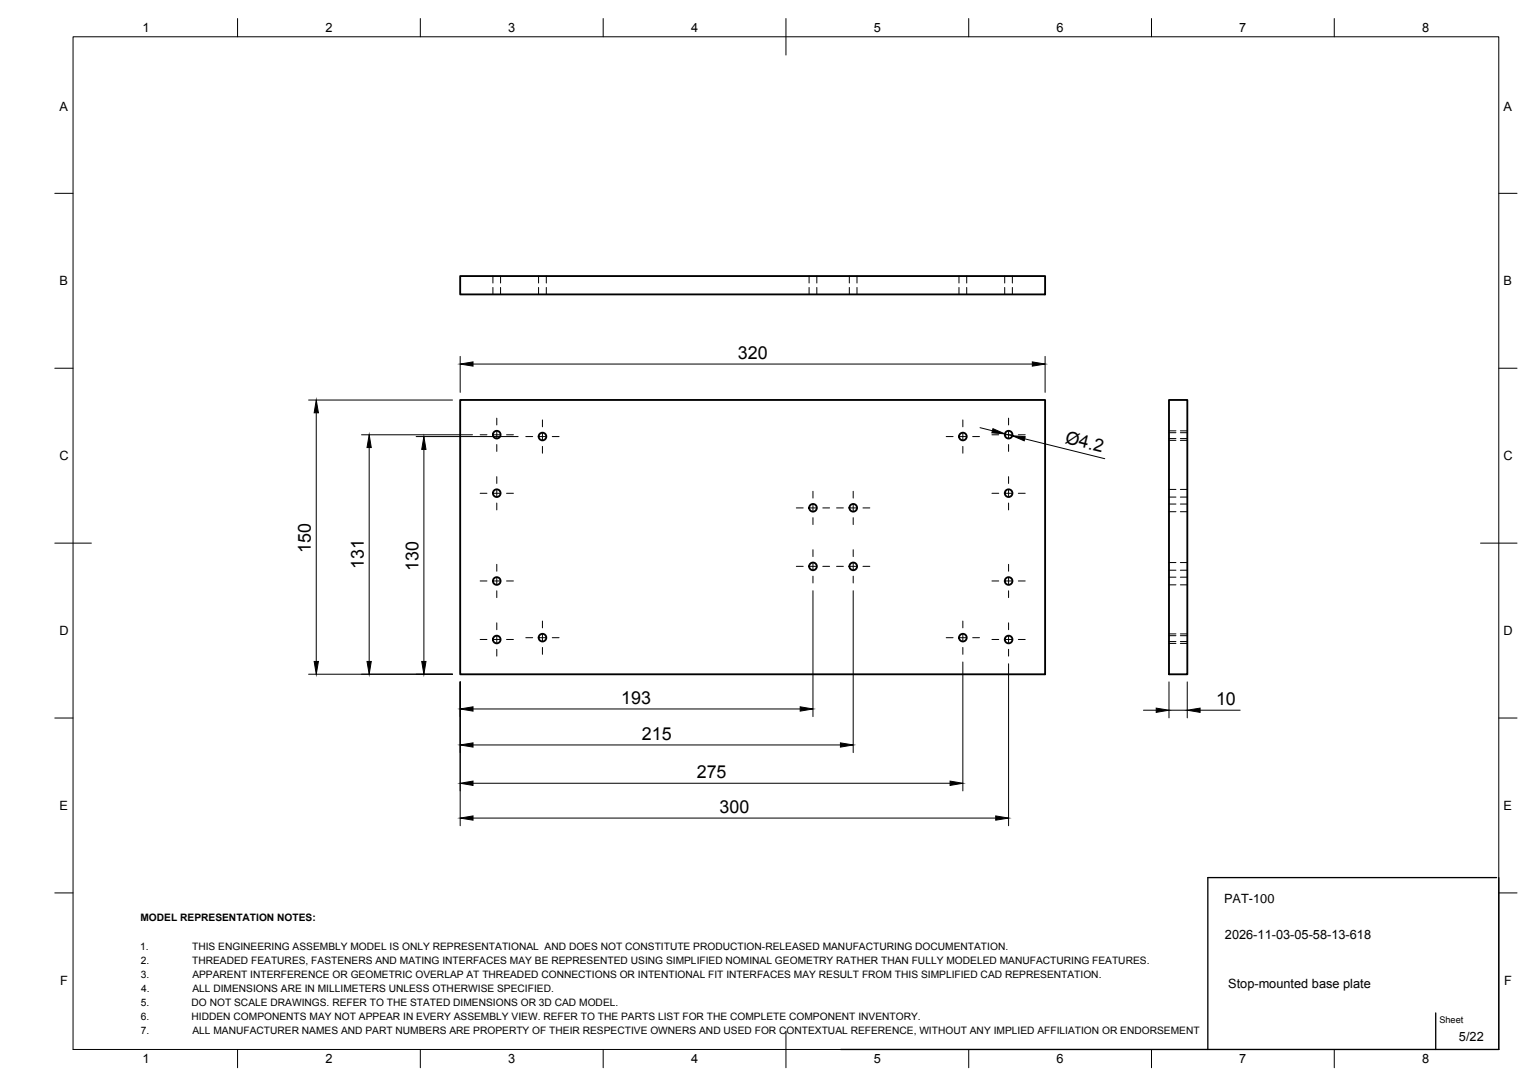
ISO-10303-21;
HEADER;
/* Generated by software containing ST-Developer
 * from STEP Tools, Inc. (www.steptools.com) 
 */

FILE_DESCRIPTION(
/* description */ (''),
/* implementation_level */ '2;1');

FILE_NAME(
/* name */ 'Stop-mounted base plate.step',
/* time_stamp */ '2026-10-29T16:43:51-07:00',
/* author */ (''),
/* organization */ (''),
/* preprocessor_version */ 'ST-DEVELOPER v20.2',
/* originating_system */ 'Autodesk Translation Framework v15.17.0.0',
/* authorisation */ '');

FILE_SCHEMA (('AUTOMOTIVE_DESIGN { 1 0 10303 214 3 1 1 }'));
ENDSEC;

DATA;
#10=MECHANICAL_DESIGN_GEOMETRIC_PRESENTATION_REPRESENTATION('',(#365),#10292);
#319=SHAPE_REPRESENTATION_RELATIONSHIP('SRR','None',#10415,#342);
#342=ADVANCED_BREP_SHAPE_REPRESENTATION('',(#388),#10267);
#365=STYLED_ITEM('',(#10607),#388);
#388=MANIFOLD_SOLID_BREP('Body1',#5007);
#406=FACE_BOUND('',#1019,.T.);
#407=FACE_BOUND('',#1020,.T.);
#408=FACE_BOUND('',#1021,.T.);
#409=FACE_BOUND('',#1022,.T.);
#410=FACE_BOUND('',#1023,.T.);
#411=FACE_BOUND('',#1024,.T.);
#412=FACE_BOUND('',#1025,.T.);
#413=FACE_BOUND('',#1026,.T.);
#414=FACE_BOUND('',#1027,.T.);
#415=FACE_BOUND('',#1028,.T.);
#416=FACE_BOUND('',#1029,.T.);
#417=FACE_BOUND('',#1030,.T.);
#418=FACE_BOUND('',#1031,.T.);
#419=FACE_BOUND('',#1032,.T.);
#420=FACE_BOUND('',#1033,.T.);
#421=FACE_BOUND('',#1034,.T.);
#422=FACE_BOUND('',#1036,.T.);
#423=FACE_BOUND('',#1037,.T.);
#424=FACE_BOUND('',#1038,.T.);
#425=FACE_BOUND('',#1039,.T.);
#426=FACE_BOUND('',#1040,.T.);
#427=FACE_BOUND('',#1041,.T.);
#428=FACE_BOUND('',#1042,.T.);
#429=FACE_BOUND('',#1043,.T.);
#430=FACE_BOUND('',#1044,.T.);
#431=FACE_BOUND('',#1045,.T.);
#432=FACE_BOUND('',#1046,.T.);
#433=FACE_BOUND('',#1047,.T.);
#434=FACE_BOUND('',#1048,.T.);
#435=FACE_BOUND('',#1049,.T.);
#436=FACE_BOUND('',#1050,.T.);
#437=FACE_BOUND('',#1051,.T.);
#531=PLANE('',#5340);
#532=PLANE('',#5341);
#533=PLANE('',#5342);
#534=PLANE('',#5343);
#535=PLANE('',#5344);
#536=PLANE('',#5345);
#710=FACE_OUTER_BOUND('',#998,.T.);
#711=FACE_OUTER_BOUND('',#999,.T.);
#712=FACE_OUTER_BOUND('',#1000,.T.);
#713=FACE_OUTER_BOUND('',#1001,.T.);
#714=FACE_OUTER_BOUND('',#1002,.T.);
#715=FACE_OUTER_BOUND('',#1003,.T.);
#716=FACE_OUTER_BOUND('',#1004,.T.);
#717=FACE_OUTER_BOUND('',#1005,.T.);
#718=FACE_OUTER_BOUND('',#1006,.T.);
#719=FACE_OUTER_BOUND('',#1007,.T.);
#720=FACE_OUTER_BOUND('',#1008,.T.);
#721=FACE_OUTER_BOUND('',#1009,.T.);
#722=FACE_OUTER_BOUND('',#1010,.T.);
#723=FACE_OUTER_BOUND('',#1011,.T.);
#724=FACE_OUTER_BOUND('',#1012,.T.);
#725=FACE_OUTER_BOUND('',#1013,.T.);
#726=FACE_OUTER_BOUND('',#1014,.T.);
#727=FACE_OUTER_BOUND('',#1015,.T.);
#728=FACE_OUTER_BOUND('',#1016,.T.);
#729=FACE_OUTER_BOUND('',#1017,.T.);
#730=FACE_OUTER_BOUND('',#1018,.T.);
#731=FACE_OUTER_BOUND('',#1035,.T.);
#998=EDGE_LOOP('',(#3409,#3410,#3411,#3412));
#999=EDGE_LOOP('',(#3413,#3414,#3415,#3416));
#1000=EDGE_LOOP('',(#3417,#3418,#3419,#3420));
#1001=EDGE_LOOP('',(#3421,#3422,#3423,#3424));
#1002=EDGE_LOOP('',(#3425,#3426,#3427,#3428));
#1003=EDGE_LOOP('',(#3429,#3430,#3431,#3432));
#1004=EDGE_LOOP('',(#3433,#3434,#3435,#3436));
#1005=EDGE_LOOP('',(#3437,#3438,#3439,#3440));
#1006=EDGE_LOOP('',(#3441,#3442,#3443,#3444));
#1007=EDGE_LOOP('',(#3445,#3446,#3447,#3448));
#1008=EDGE_LOOP('',(#3449,#3450,#3451,#3452));
#1009=EDGE_LOOP('',(#3453,#3454,#3455,#3456));
#1010=EDGE_LOOP('',(#3457,#3458,#3459,#3460));
#1011=EDGE_LOOP('',(#3461,#3462,#3463,#3464));
#1012=EDGE_LOOP('',(#3465,#3466,#3467,#3468));
#1013=EDGE_LOOP('',(#3469,#3470,#3471,#3472));
#1014=EDGE_LOOP('',(#3473,#3474,#3475,#3476));
#1015=EDGE_LOOP('',(#3477,#3478,#3479,#3480));
#1016=EDGE_LOOP('',(#3481,#3482,#3483,#3484));
#1017=EDGE_LOOP('',(#3485,#3486,#3487,#3488));
#1018=EDGE_LOOP('',(#3489,#3490,#3491,#3492));
#1019=EDGE_LOOP('',(#3493));
#1020=EDGE_LOOP('',(#3494));
#1021=EDGE_LOOP('',(#3495));
#1022=EDGE_LOOP('',(#3496));
#1023=EDGE_LOOP('',(#3497));
#1024=EDGE_LOOP('',(#3498));
#1025=EDGE_LOOP('',(#3499));
#1026=EDGE_LOOP('',(#3500));
#1027=EDGE_LOOP('',(#3501));
#1028=EDGE_LOOP('',(#3502));
#1029=EDGE_LOOP('',(#3503));
#1030=EDGE_LOOP('',(#3504));
#1031=EDGE_LOOP('',(#3505));
#1032=EDGE_LOOP('',(#3506));
#1033=EDGE_LOOP('',(#3507));
#1034=EDGE_LOOP('',(#3508));
#1035=EDGE_LOOP('',(#3509,#3510,#3511,#3512));
#1036=EDGE_LOOP('',(#3513));
#1037=EDGE_LOOP('',(#3514));
#1038=EDGE_LOOP('',(#3515));
#1039=EDGE_LOOP('',(#3516));
#1040=EDGE_LOOP('',(#3517));
#1041=EDGE_LOOP('',(#3518));
#1042=EDGE_LOOP('',(#3519));
#1043=EDGE_LOOP('',(#3520));
#1044=EDGE_LOOP('',(#3521));
#1045=EDGE_LOOP('',(#3522));
#1046=EDGE_LOOP('',(#3523));
#1047=EDGE_LOOP('',(#3524));
#1048=EDGE_LOOP('',(#3525));
#1049=EDGE_LOOP('',(#3526));
#1050=EDGE_LOOP('',(#3527));
#1051=EDGE_LOOP('',(#3528));
#1411=LINE('',#7413,#1803);
#1412=LINE('',#7419,#1804);
#1413=LINE('',#7425,#1805);
#1414=LINE('',#7431,#1806);
#1415=LINE('',#7437,#1807);
#1416=LINE('',#7443,#1808);
#1417=LINE('',#7449,#1809);
#1418=LINE('',#7455,#1810);
#1419=LINE('',#7461,#1811);
#1420=LINE('',#7467,#1812);
#1421=LINE('',#7473,#1813);
#1422=LINE('',#7479,#1814);
#1423=LINE('',#7485,#1815);
#1424=LINE('',#7491,#1816);
#1425=LINE('',#7497,#1817);
#1426=LINE('',#7503,#1818);
#1427=LINE('',#7508,#1819);
#1428=LINE('',#7510,#1820);
#1429=LINE('',#7512,#1821);
#1430=LINE('',#7513,#1822);
#1431=LINE('',#7516,#1823);
#1432=LINE('',#7518,#1824);
#1433=LINE('',#7519,#1825);
#1434=LINE('',#7522,#1826);
#1435=LINE('',#7524,#1827);
#1436=LINE('',#7525,#1828);
#1437=LINE('',#7527,#1829);
#1438=LINE('',#7528,#1830);
#1803=VECTOR('',#5874,0.210000000000001);
#1804=VECTOR('',#5881,0.210000000000001);
#1805=VECTOR('',#5888,0.210000000000001);
#1806=VECTOR('',#5895,0.210000000000001);
#1807=VECTOR('',#5902,0.210000000000001);
#1808=VECTOR('',#5909,0.21);
#1809=VECTOR('',#5916,0.21);
#1810=VECTOR('',#5923,0.210000000000001);
#1811=VECTOR('',#5930,0.210000000000001);
#1812=VECTOR('',#5937,0.210000000000001);
#1813=VECTOR('',#5944,0.21);
#1814=VECTOR('',#5951,0.21);
#1815=VECTOR('',#5958,0.21);
#1816=VECTOR('',#5965,0.21);
#1817=VECTOR('',#5972,0.210000000000001);
#1818=VECTOR('',#5979,0.210000000000001);
#1819=VECTOR('',#5984,1.);
#1820=VECTOR('',#5985,1.);
#1821=VECTOR('',#5986,1.);
#1822=VECTOR('',#5987,1.);
#1823=VECTOR('',#5990,1.);
#1824=VECTOR('',#5991,1.);
#1825=VECTOR('',#5992,1.);
#1826=VECTOR('',#5995,1.);
#1827=VECTOR('',#5996,1.);
#1828=VECTOR('',#5997,1.);
#1829=VECTOR('',#6000,1.);
#1830=VECTOR('',#6001,1.);
#2195=CIRCLE('',#5293,0.210000000000001);
#2196=CIRCLE('',#5294,0.210000000000001);
#2197=CIRCLE('',#5296,0.210000000000001);
#2198=CIRCLE('',#5297,0.210000000000001);
#2199=CIRCLE('',#5299,0.210000000000001);
#2200=CIRCLE('',#5300,0.210000000000001);
#2201=CIRCLE('',#5302,0.210000000000001);
#2202=CIRCLE('',#5303,0.210000000000001);
#2203=CIRCLE('',#5305,0.210000000000001);
#2204=CIRCLE('',#5306,0.210000000000001);
#2205=CIRCLE('',#5308,0.21);
#2206=CIRCLE('',#5309,0.21);
#2207=CIRCLE('',#5311,0.21);
#2208=CIRCLE('',#5312,0.21);
#2209=CIRCLE('',#5314,0.210000000000001);
#2210=CIRCLE('',#5315,0.210000000000001);
#2211=CIRCLE('',#5317,0.210000000000001);
#2212=CIRCLE('',#5318,0.210000000000001);
#2213=CIRCLE('',#5320,0.210000000000001);
#2214=CIRCLE('',#5321,0.210000000000001);
#2215=CIRCLE('',#5323,0.21);
#2216=CIRCLE('',#5324,0.21);
#2217=CIRCLE('',#5326,0.21);
#2218=CIRCLE('',#5327,0.21);
#2219=CIRCLE('',#5329,0.21);
#2220=CIRCLE('',#5330,0.21);
#2221=CIRCLE('',#5332,0.21);
#2222=CIRCLE('',#5333,0.21);
#2223=CIRCLE('',#5335,0.210000000000001);
#2224=CIRCLE('',#5336,0.210000000000001);
#2225=CIRCLE('',#5338,0.210000000000001);
#2226=CIRCLE('',#5339,0.210000000000001);
#2394=VERTEX_POINT('',#7410);
#2395=VERTEX_POINT('',#7412);
#2396=VERTEX_POINT('',#7416);
#2397=VERTEX_POINT('',#7418);
#2398=VERTEX_POINT('',#7422);
#2399=VERTEX_POINT('',#7424);
#2400=VERTEX_POINT('',#7428);
#2401=VERTEX_POINT('',#7430);
#2402=VERTEX_POINT('',#7434);
#2403=VERTEX_POINT('',#7436);
#2404=VERTEX_POINT('',#7440);
#2405=VERTEX_POINT('',#7442);
#2406=VERTEX_POINT('',#7446);
#2407=VERTEX_POINT('',#7448);
#2408=VERTEX_POINT('',#7452);
#2409=VERTEX_POINT('',#7454);
#2410=VERTEX_POINT('',#7458);
#2411=VERTEX_POINT('',#7460);
#2412=VERTEX_POINT('',#7464);
#2413=VERTEX_POINT('',#7466);
#2414=VERTEX_POINT('',#7470);
#2415=VERTEX_POINT('',#7472);
#2416=VERTEX_POINT('',#7476);
#2417=VERTEX_POINT('',#7478);
#2418=VERTEX_POINT('',#7482);
#2419=VERTEX_POINT('',#7484);
#2420=VERTEX_POINT('',#7488);
#2421=VERTEX_POINT('',#7490);
#2422=VERTEX_POINT('',#7494);
#2423=VERTEX_POINT('',#7496);
#2424=VERTEX_POINT('',#7500);
#2425=VERTEX_POINT('',#7502);
#2426=VERTEX_POINT('',#7506);
#2427=VERTEX_POINT('',#7507);
#2428=VERTEX_POINT('',#7509);
#2429=VERTEX_POINT('',#7511);
#2430=VERTEX_POINT('',#7515);
#2431=VERTEX_POINT('',#7517);
#2432=VERTEX_POINT('',#7521);
#2433=VERTEX_POINT('',#7523);
#2795=EDGE_CURVE('',#2394,#2394,#2195,.T.);
#2796=EDGE_CURVE('',#2394,#2395,#1411,.T.);
#2797=EDGE_CURVE('',#2395,#2395,#2196,.T.);
#2798=EDGE_CURVE('',#2396,#2396,#2197,.T.);
#2799=EDGE_CURVE('',#2396,#2397,#1412,.T.);
#2800=EDGE_CURVE('',#2397,#2397,#2198,.T.);
#2801=EDGE_CURVE('',#2398,#2398,#2199,.T.);
#2802=EDGE_CURVE('',#2398,#2399,#1413,.T.);
#2803=EDGE_CURVE('',#2399,#2399,#2200,.T.);
#2804=EDGE_CURVE('',#2400,#2400,#2201,.T.);
#2805=EDGE_CURVE('',#2400,#2401,#1414,.T.);
#2806=EDGE_CURVE('',#2401,#2401,#2202,.T.);
#2807=EDGE_CURVE('',#2402,#2402,#2203,.T.);
#2808=EDGE_CURVE('',#2402,#2403,#1415,.T.);
#2809=EDGE_CURVE('',#2403,#2403,#2204,.T.);
#2810=EDGE_CURVE('',#2404,#2404,#2205,.T.);
#2811=EDGE_CURVE('',#2404,#2405,#1416,.T.);
#2812=EDGE_CURVE('',#2405,#2405,#2206,.T.);
#2813=EDGE_CURVE('',#2406,#2406,#2207,.T.);
#2814=EDGE_CURVE('',#2406,#2407,#1417,.T.);
#2815=EDGE_CURVE('',#2407,#2407,#2208,.T.);
#2816=EDGE_CURVE('',#2408,#2408,#2209,.T.);
#2817=EDGE_CURVE('',#2408,#2409,#1418,.T.);
#2818=EDGE_CURVE('',#2409,#2409,#2210,.T.);
#2819=EDGE_CURVE('',#2410,#2410,#2211,.T.);
#2820=EDGE_CURVE('',#2410,#2411,#1419,.T.);
#2821=EDGE_CURVE('',#2411,#2411,#2212,.T.);
#2822=EDGE_CURVE('',#2412,#2412,#2213,.T.);
#2823=EDGE_CURVE('',#2412,#2413,#1420,.T.);
#2824=EDGE_CURVE('',#2413,#2413,#2214,.T.);
#2825=EDGE_CURVE('',#2414,#2414,#2215,.T.);
#2826=EDGE_CURVE('',#2414,#2415,#1421,.T.);
#2827=EDGE_CURVE('',#2415,#2415,#2216,.T.);
#2828=EDGE_CURVE('',#2416,#2416,#2217,.T.);
#2829=EDGE_CURVE('',#2416,#2417,#1422,.T.);
#2830=EDGE_CURVE('',#2417,#2417,#2218,.T.);
#2831=EDGE_CURVE('',#2418,#2418,#2219,.T.);
#2832=EDGE_CURVE('',#2418,#2419,#1423,.T.);
#2833=EDGE_CURVE('',#2419,#2419,#2220,.T.);
#2834=EDGE_CURVE('',#2420,#2420,#2221,.T.);
#2835=EDGE_CURVE('',#2420,#2421,#1424,.T.);
#2836=EDGE_CURVE('',#2421,#2421,#2222,.T.);
#2837=EDGE_CURVE('',#2422,#2422,#2223,.T.);
#2838=EDGE_CURVE('',#2422,#2423,#1425,.T.);
#2839=EDGE_CURVE('',#2423,#2423,#2224,.T.);
#2840=EDGE_CURVE('',#2424,#2424,#2225,.T.);
#2841=EDGE_CURVE('',#2424,#2425,#1426,.T.);
#2842=EDGE_CURVE('',#2425,#2425,#2226,.T.);
#2843=EDGE_CURVE('',#2426,#2427,#1427,.T.);
#2844=EDGE_CURVE('',#2427,#2428,#1428,.T.);
#2845=EDGE_CURVE('',#2429,#2428,#1429,.T.);
#2846=EDGE_CURVE('',#2426,#2429,#1430,.T.);
#2847=EDGE_CURVE('',#2430,#2426,#1431,.T.);
#2848=EDGE_CURVE('',#2431,#2429,#1432,.T.);
#2849=EDGE_CURVE('',#2430,#2431,#1433,.T.);
#2850=EDGE_CURVE('',#2432,#2430,#1434,.T.);
#2851=EDGE_CURVE('',#2433,#2431,#1435,.T.);
#2852=EDGE_CURVE('',#2432,#2433,#1436,.T.);
#2853=EDGE_CURVE('',#2427,#2432,#1437,.T.);
#2854=EDGE_CURVE('',#2428,#2433,#1438,.T.);
#3409=ORIENTED_EDGE('',*,*,#2795,.F.);
#3410=ORIENTED_EDGE('',*,*,#2796,.T.);
#3411=ORIENTED_EDGE('',*,*,#2797,.F.);
#3412=ORIENTED_EDGE('',*,*,#2796,.F.);
#3413=ORIENTED_EDGE('',*,*,#2798,.F.);
#3414=ORIENTED_EDGE('',*,*,#2799,.T.);
#3415=ORIENTED_EDGE('',*,*,#2800,.F.);
#3416=ORIENTED_EDGE('',*,*,#2799,.F.);
#3417=ORIENTED_EDGE('',*,*,#2801,.F.);
#3418=ORIENTED_EDGE('',*,*,#2802,.T.);
#3419=ORIENTED_EDGE('',*,*,#2803,.F.);
#3420=ORIENTED_EDGE('',*,*,#2802,.F.);
#3421=ORIENTED_EDGE('',*,*,#2804,.F.);
#3422=ORIENTED_EDGE('',*,*,#2805,.T.);
#3423=ORIENTED_EDGE('',*,*,#2806,.F.);
#3424=ORIENTED_EDGE('',*,*,#2805,.F.);
#3425=ORIENTED_EDGE('',*,*,#2807,.F.);
#3426=ORIENTED_EDGE('',*,*,#2808,.T.);
#3427=ORIENTED_EDGE('',*,*,#2809,.F.);
#3428=ORIENTED_EDGE('',*,*,#2808,.F.);
#3429=ORIENTED_EDGE('',*,*,#2810,.F.);
#3430=ORIENTED_EDGE('',*,*,#2811,.T.);
#3431=ORIENTED_EDGE('',*,*,#2812,.F.);
#3432=ORIENTED_EDGE('',*,*,#2811,.F.);
#3433=ORIENTED_EDGE('',*,*,#2813,.F.);
#3434=ORIENTED_EDGE('',*,*,#2814,.T.);
#3435=ORIENTED_EDGE('',*,*,#2815,.F.);
#3436=ORIENTED_EDGE('',*,*,#2814,.F.);
#3437=ORIENTED_EDGE('',*,*,#2816,.F.);
#3438=ORIENTED_EDGE('',*,*,#2817,.T.);
#3439=ORIENTED_EDGE('',*,*,#2818,.F.);
#3440=ORIENTED_EDGE('',*,*,#2817,.F.);
#3441=ORIENTED_EDGE('',*,*,#2819,.F.);
#3442=ORIENTED_EDGE('',*,*,#2820,.T.);
#3443=ORIENTED_EDGE('',*,*,#2821,.F.);
#3444=ORIENTED_EDGE('',*,*,#2820,.F.);
#3445=ORIENTED_EDGE('',*,*,#2822,.F.);
#3446=ORIENTED_EDGE('',*,*,#2823,.T.);
#3447=ORIENTED_EDGE('',*,*,#2824,.F.);
#3448=ORIENTED_EDGE('',*,*,#2823,.F.);
#3449=ORIENTED_EDGE('',*,*,#2825,.F.);
#3450=ORIENTED_EDGE('',*,*,#2826,.T.);
#3451=ORIENTED_EDGE('',*,*,#2827,.F.);
#3452=ORIENTED_EDGE('',*,*,#2826,.F.);
#3453=ORIENTED_EDGE('',*,*,#2828,.F.);
#3454=ORIENTED_EDGE('',*,*,#2829,.T.);
#3455=ORIENTED_EDGE('',*,*,#2830,.F.);
#3456=ORIENTED_EDGE('',*,*,#2829,.F.);
#3457=ORIENTED_EDGE('',*,*,#2831,.F.);
#3458=ORIENTED_EDGE('',*,*,#2832,.T.);
#3459=ORIENTED_EDGE('',*,*,#2833,.F.);
#3460=ORIENTED_EDGE('',*,*,#2832,.F.);
#3461=ORIENTED_EDGE('',*,*,#2834,.F.);
#3462=ORIENTED_EDGE('',*,*,#2835,.T.);
#3463=ORIENTED_EDGE('',*,*,#2836,.F.);
#3464=ORIENTED_EDGE('',*,*,#2835,.F.);
#3465=ORIENTED_EDGE('',*,*,#2837,.F.);
#3466=ORIENTED_EDGE('',*,*,#2838,.T.);
#3467=ORIENTED_EDGE('',*,*,#2839,.F.);
#3468=ORIENTED_EDGE('',*,*,#2838,.F.);
#3469=ORIENTED_EDGE('',*,*,#2840,.F.);
#3470=ORIENTED_EDGE('',*,*,#2841,.T.);
#3471=ORIENTED_EDGE('',*,*,#2842,.F.);
#3472=ORIENTED_EDGE('',*,*,#2841,.F.);
#3473=ORIENTED_EDGE('',*,*,#2843,.T.);
#3474=ORIENTED_EDGE('',*,*,#2844,.T.);
#3475=ORIENTED_EDGE('',*,*,#2845,.F.);
#3476=ORIENTED_EDGE('',*,*,#2846,.F.);
#3477=ORIENTED_EDGE('',*,*,#2847,.T.);
#3478=ORIENTED_EDGE('',*,*,#2846,.T.);
#3479=ORIENTED_EDGE('',*,*,#2848,.F.);
#3480=ORIENTED_EDGE('',*,*,#2849,.F.);
#3481=ORIENTED_EDGE('',*,*,#2850,.T.);
#3482=ORIENTED_EDGE('',*,*,#2849,.T.);
#3483=ORIENTED_EDGE('',*,*,#2851,.F.);
#3484=ORIENTED_EDGE('',*,*,#2852,.F.);
#3485=ORIENTED_EDGE('',*,*,#2853,.T.);
#3486=ORIENTED_EDGE('',*,*,#2852,.T.);
#3487=ORIENTED_EDGE('',*,*,#2854,.F.);
#3488=ORIENTED_EDGE('',*,*,#2844,.F.);
#3489=ORIENTED_EDGE('',*,*,#2854,.T.);
#3490=ORIENTED_EDGE('',*,*,#2851,.T.);
#3491=ORIENTED_EDGE('',*,*,#2848,.T.);
#3492=ORIENTED_EDGE('',*,*,#2845,.T.);
#3493=ORIENTED_EDGE('',*,*,#2809,.T.);
#3494=ORIENTED_EDGE('',*,*,#2812,.T.);
#3495=ORIENTED_EDGE('',*,*,#2815,.T.);
#3496=ORIENTED_EDGE('',*,*,#2818,.T.);
#3497=ORIENTED_EDGE('',*,*,#2842,.T.);
#3498=ORIENTED_EDGE('',*,*,#2839,.T.);
#3499=ORIENTED_EDGE('',*,*,#2836,.T.);
#3500=ORIENTED_EDGE('',*,*,#2833,.T.);
#3501=ORIENTED_EDGE('',*,*,#2830,.T.);
#3502=ORIENTED_EDGE('',*,*,#2827,.T.);
#3503=ORIENTED_EDGE('',*,*,#2824,.T.);
#3504=ORIENTED_EDGE('',*,*,#2821,.T.);
#3505=ORIENTED_EDGE('',*,*,#2806,.T.);
#3506=ORIENTED_EDGE('',*,*,#2803,.T.);
#3507=ORIENTED_EDGE('',*,*,#2800,.T.);
#3508=ORIENTED_EDGE('',*,*,#2797,.T.);
#3509=ORIENTED_EDGE('',*,*,#2853,.F.);
#3510=ORIENTED_EDGE('',*,*,#2843,.F.);
#3511=ORIENTED_EDGE('',*,*,#2847,.F.);
#3512=ORIENTED_EDGE('',*,*,#2850,.F.);
#3513=ORIENTED_EDGE('',*,*,#2807,.T.);
#3514=ORIENTED_EDGE('',*,*,#2810,.T.);
#3515=ORIENTED_EDGE('',*,*,#2813,.T.);
#3516=ORIENTED_EDGE('',*,*,#2816,.T.);
#3517=ORIENTED_EDGE('',*,*,#2840,.T.);
#3518=ORIENTED_EDGE('',*,*,#2837,.T.);
#3519=ORIENTED_EDGE('',*,*,#2834,.T.);
#3520=ORIENTED_EDGE('',*,*,#2831,.T.);
#3521=ORIENTED_EDGE('',*,*,#2828,.T.);
#3522=ORIENTED_EDGE('',*,*,#2825,.T.);
#3523=ORIENTED_EDGE('',*,*,#2822,.T.);
#3524=ORIENTED_EDGE('',*,*,#2819,.T.);
#3525=ORIENTED_EDGE('',*,*,#2804,.T.);
#3526=ORIENTED_EDGE('',*,*,#2801,.T.);
#3527=ORIENTED_EDGE('',*,*,#2798,.T.);
#3528=ORIENTED_EDGE('',*,*,#2795,.T.);
#4637=CYLINDRICAL_SURFACE('',#5292,0.210000000000001);
#4638=CYLINDRICAL_SURFACE('',#5295,0.210000000000001);
#4639=CYLINDRICAL_SURFACE('',#5298,0.210000000000001);
#4640=CYLINDRICAL_SURFACE('',#5301,0.210000000000001);
#4641=CYLINDRICAL_SURFACE('',#5304,0.210000000000001);
#4642=CYLINDRICAL_SURFACE('',#5307,0.21);
#4643=CYLINDRICAL_SURFACE('',#5310,0.21);
#4644=CYLINDRICAL_SURFACE('',#5313,0.210000000000001);
#4645=CYLINDRICAL_SURFACE('',#5316,0.210000000000001);
#4646=CYLINDRICAL_SURFACE('',#5319,0.210000000000001);
#4647=CYLINDRICAL_SURFACE('',#5322,0.21);
#4648=CYLINDRICAL_SURFACE('',#5325,0.21);
#4649=CYLINDRICAL_SURFACE('',#5328,0.21);
#4650=CYLINDRICAL_SURFACE('',#5331,0.21);
#4651=CYLINDRICAL_SURFACE('',#5334,0.210000000000001);
#4652=CYLINDRICAL_SURFACE('',#5337,0.210000000000001);
#4719=ADVANCED_FACE('',(#710),#4637,.F.);
#4720=ADVANCED_FACE('',(#711),#4638,.F.);
#4721=ADVANCED_FACE('',(#712),#4639,.F.);
#4722=ADVANCED_FACE('',(#713),#4640,.F.);
#4723=ADVANCED_FACE('',(#714),#4641,.F.);
#4724=ADVANCED_FACE('',(#715),#4642,.F.);
#4725=ADVANCED_FACE('',(#716),#4643,.F.);
#4726=ADVANCED_FACE('',(#717),#4644,.F.);
#4727=ADVANCED_FACE('',(#718),#4645,.F.);
#4728=ADVANCED_FACE('',(#719),#4646,.F.);
#4729=ADVANCED_FACE('',(#720),#4647,.F.);
#4730=ADVANCED_FACE('',(#721),#4648,.F.);
#4731=ADVANCED_FACE('',(#722),#4649,.F.);
#4732=ADVANCED_FACE('',(#723),#4650,.F.);
#4733=ADVANCED_FACE('',(#724),#4651,.F.);
#4734=ADVANCED_FACE('',(#725),#4652,.F.);
#4735=ADVANCED_FACE('',(#726),#531,.T.);
#4736=ADVANCED_FACE('',(#727),#532,.T.);
#4737=ADVANCED_FACE('',(#728),#533,.T.);
#4738=ADVANCED_FACE('',(#729),#534,.T.);
#4739=ADVANCED_FACE('',(#730,#406,#407,#408,#409,#410,#411,#412,#413,#414,
#415,#416,#417,#418,#419,#420,#421),#535,.T.);
#4740=ADVANCED_FACE('',(#731,#422,#423,#424,#425,#426,#427,#428,#429,#430,
#431,#432,#433,#434,#435,#436,#437),#536,.F.);
#5007=CLOSED_SHELL('',(#4719,#4720,#4721,#4722,#4723,#4724,#4725,#4726,
#4727,#4728,#4729,#4730,#4731,#4732,#4733,#4734,#4735,#4736,#4737,#4738,
#4739,#4740));
#5291=AXIS2_PLACEMENT_3D('',#7408,#5868,#5869);
#5292=AXIS2_PLACEMENT_3D('',#7409,#5870,#5871);
#5293=AXIS2_PLACEMENT_3D('',#7411,#5872,#5873);
#5294=AXIS2_PLACEMENT_3D('',#7414,#5875,#5876);
#5295=AXIS2_PLACEMENT_3D('',#7415,#5877,#5878);
#5296=AXIS2_PLACEMENT_3D('',#7417,#5879,#5880);
#5297=AXIS2_PLACEMENT_3D('',#7420,#5882,#5883);
#5298=AXIS2_PLACEMENT_3D('',#7421,#5884,#5885);
#5299=AXIS2_PLACEMENT_3D('',#7423,#5886,#5887);
#5300=AXIS2_PLACEMENT_3D('',#7426,#5889,#5890);
#5301=AXIS2_PLACEMENT_3D('',#7427,#5891,#5892);
#5302=AXIS2_PLACEMENT_3D('',#7429,#5893,#5894);
#5303=AXIS2_PLACEMENT_3D('',#7432,#5896,#5897);
#5304=AXIS2_PLACEMENT_3D('',#7433,#5898,#5899);
#5305=AXIS2_PLACEMENT_3D('',#7435,#5900,#5901);
#5306=AXIS2_PLACEMENT_3D('',#7438,#5903,#5904);
#5307=AXIS2_PLACEMENT_3D('',#7439,#5905,#5906);
#5308=AXIS2_PLACEMENT_3D('',#7441,#5907,#5908);
#5309=AXIS2_PLACEMENT_3D('',#7444,#5910,#5911);
#5310=AXIS2_PLACEMENT_3D('',#7445,#5912,#5913);
#5311=AXIS2_PLACEMENT_3D('',#7447,#5914,#5915);
#5312=AXIS2_PLACEMENT_3D('',#7450,#5917,#5918);
#5313=AXIS2_PLACEMENT_3D('',#7451,#5919,#5920);
#5314=AXIS2_PLACEMENT_3D('',#7453,#5921,#5922);
#5315=AXIS2_PLACEMENT_3D('',#7456,#5924,#5925);
#5316=AXIS2_PLACEMENT_3D('',#7457,#5926,#5927);
#5317=AXIS2_PLACEMENT_3D('',#7459,#5928,#5929);
#5318=AXIS2_PLACEMENT_3D('',#7462,#5931,#5932);
#5319=AXIS2_PLACEMENT_3D('',#7463,#5933,#5934);
#5320=AXIS2_PLACEMENT_3D('',#7465,#5935,#5936);
#5321=AXIS2_PLACEMENT_3D('',#7468,#5938,#5939);
#5322=AXIS2_PLACEMENT_3D('',#7469,#5940,#5941);
#5323=AXIS2_PLACEMENT_3D('',#7471,#5942,#5943);
#5324=AXIS2_PLACEMENT_3D('',#7474,#5945,#5946);
#5325=AXIS2_PLACEMENT_3D('',#7475,#5947,#5948);
#5326=AXIS2_PLACEMENT_3D('',#7477,#5949,#5950);
#5327=AXIS2_PLACEMENT_3D('',#7480,#5952,#5953);
#5328=AXIS2_PLACEMENT_3D('',#7481,#5954,#5955);
#5329=AXIS2_PLACEMENT_3D('',#7483,#5956,#5957);
#5330=AXIS2_PLACEMENT_3D('',#7486,#5959,#5960);
#5331=AXIS2_PLACEMENT_3D('',#7487,#5961,#5962);
#5332=AXIS2_PLACEMENT_3D('',#7489,#5963,#5964);
#5333=AXIS2_PLACEMENT_3D('',#7492,#5966,#5967);
#5334=AXIS2_PLACEMENT_3D('',#7493,#5968,#5969);
#5335=AXIS2_PLACEMENT_3D('',#7495,#5970,#5971);
#5336=AXIS2_PLACEMENT_3D('',#7498,#5973,#5974);
#5337=AXIS2_PLACEMENT_3D('',#7499,#5975,#5976);
#5338=AXIS2_PLACEMENT_3D('',#7501,#5977,#5978);
#5339=AXIS2_PLACEMENT_3D('',#7504,#5980,#5981);
#5340=AXIS2_PLACEMENT_3D('',#7505,#5982,#5983);
#5341=AXIS2_PLACEMENT_3D('',#7514,#5988,#5989);
#5342=AXIS2_PLACEMENT_3D('',#7520,#5993,#5994);
#5343=AXIS2_PLACEMENT_3D('',#7526,#5998,#5999);
#5344=AXIS2_PLACEMENT_3D('',#7529,#6002,#6003);
#5345=AXIS2_PLACEMENT_3D('',#7530,#6004,#6005);
#5868=DIRECTION('axis',(0.,0.,1.));
#5869=DIRECTION('refdir',(1.,0.,0.));
#5870=DIRECTION('center_axis',(0.,0.,1.));
#5871=DIRECTION('ref_axis',(1.,0.,0.));
#5872=DIRECTION('center_axis',(0.,0.,1.));
#5873=DIRECTION('ref_axis',(1.,0.,0.));
#5874=DIRECTION('',(0.,0.,1.));
#5875=DIRECTION('center_axis',(0.,0.,-1.));
#5876=DIRECTION('ref_axis',(1.,0.,0.));
#5877=DIRECTION('center_axis',(0.,0.,1.));
#5878=DIRECTION('ref_axis',(1.,0.,0.));
#5879=DIRECTION('center_axis',(0.,0.,1.));
#5880=DIRECTION('ref_axis',(1.,0.,0.));
#5881=DIRECTION('',(0.,0.,1.));
#5882=DIRECTION('center_axis',(0.,0.,-1.));
#5883=DIRECTION('ref_axis',(1.,0.,0.));
#5884=DIRECTION('center_axis',(0.,0.,1.));
#5885=DIRECTION('ref_axis',(1.,0.,0.));
#5886=DIRECTION('center_axis',(0.,0.,1.));
#5887=DIRECTION('ref_axis',(1.,0.,0.));
#5888=DIRECTION('',(0.,0.,1.));
#5889=DIRECTION('center_axis',(0.,0.,-1.));
#5890=DIRECTION('ref_axis',(1.,0.,0.));
#5891=DIRECTION('center_axis',(0.,0.,1.));
#5892=DIRECTION('ref_axis',(1.,0.,0.));
#5893=DIRECTION('center_axis',(0.,0.,1.));
#5894=DIRECTION('ref_axis',(1.,0.,0.));
#5895=DIRECTION('',(0.,0.,1.));
#5896=DIRECTION('center_axis',(0.,0.,-1.));
#5897=DIRECTION('ref_axis',(1.,0.,0.));
#5898=DIRECTION('center_axis',(0.,0.,1.));
#5899=DIRECTION('ref_axis',(1.,0.,0.));
#5900=DIRECTION('center_axis',(0.,0.,1.));
#5901=DIRECTION('ref_axis',(1.,0.,0.));
#5902=DIRECTION('',(0.,0.,1.));
#5903=DIRECTION('center_axis',(0.,0.,-1.));
#5904=DIRECTION('ref_axis',(1.,0.,0.));
#5905=DIRECTION('center_axis',(0.,0.,1.));
#5906=DIRECTION('ref_axis',(1.,0.,0.));
#5907=DIRECTION('center_axis',(0.,0.,1.));
#5908=DIRECTION('ref_axis',(1.,0.,0.));
#5909=DIRECTION('',(0.,0.,1.));
#5910=DIRECTION('center_axis',(0.,0.,-1.));
#5911=DIRECTION('ref_axis',(1.,0.,0.));
#5912=DIRECTION('center_axis',(0.,0.,1.));
#5913=DIRECTION('ref_axis',(1.,0.,0.));
#5914=DIRECTION('center_axis',(0.,0.,1.));
#5915=DIRECTION('ref_axis',(1.,0.,0.));
#5916=DIRECTION('',(0.,0.,1.));
#5917=DIRECTION('center_axis',(0.,0.,-1.));
#5918=DIRECTION('ref_axis',(1.,0.,0.));
#5919=DIRECTION('center_axis',(0.,0.,1.));
#5920=DIRECTION('ref_axis',(1.,0.,0.));
#5921=DIRECTION('center_axis',(0.,0.,1.));
#5922=DIRECTION('ref_axis',(1.,0.,0.));
#5923=DIRECTION('',(0.,0.,1.));
#5924=DIRECTION('center_axis',(0.,0.,-1.));
#5925=DIRECTION('ref_axis',(1.,0.,0.));
#5926=DIRECTION('center_axis',(0.,0.,1.));
#5927=DIRECTION('ref_axis',(1.,0.,0.));
#5928=DIRECTION('center_axis',(0.,0.,1.));
#5929=DIRECTION('ref_axis',(1.,0.,0.));
#5930=DIRECTION('',(0.,0.,1.));
#5931=DIRECTION('center_axis',(0.,0.,-1.));
#5932=DIRECTION('ref_axis',(1.,0.,0.));
#5933=DIRECTION('center_axis',(0.,0.,1.));
#5934=DIRECTION('ref_axis',(1.,0.,0.));
#5935=DIRECTION('center_axis',(0.,0.,1.));
#5936=DIRECTION('ref_axis',(1.,0.,0.));
#5937=DIRECTION('',(0.,0.,1.));
#5938=DIRECTION('center_axis',(0.,0.,-1.));
#5939=DIRECTION('ref_axis',(1.,0.,0.));
#5940=DIRECTION('center_axis',(0.,0.,1.));
#5941=DIRECTION('ref_axis',(1.,0.,0.));
#5942=DIRECTION('center_axis',(0.,0.,1.));
#5943=DIRECTION('ref_axis',(1.,0.,0.));
#5944=DIRECTION('',(0.,0.,1.));
#5945=DIRECTION('center_axis',(0.,0.,-1.));
#5946=DIRECTION('ref_axis',(1.,0.,0.));
#5947=DIRECTION('center_axis',(0.,0.,1.));
#5948=DIRECTION('ref_axis',(1.,0.,0.));
#5949=DIRECTION('center_axis',(0.,0.,1.));
#5950=DIRECTION('ref_axis',(1.,0.,0.));
#5951=DIRECTION('',(0.,0.,1.));
#5952=DIRECTION('center_axis',(0.,0.,-1.));
#5953=DIRECTION('ref_axis',(1.,0.,0.));
#5954=DIRECTION('center_axis',(0.,0.,1.));
#5955=DIRECTION('ref_axis',(1.,0.,0.));
#5956=DIRECTION('center_axis',(0.,0.,1.));
#5957=DIRECTION('ref_axis',(1.,0.,0.));
#5958=DIRECTION('',(0.,0.,1.));
#5959=DIRECTION('center_axis',(0.,0.,-1.));
#5960=DIRECTION('ref_axis',(1.,0.,0.));
#5961=DIRECTION('center_axis',(0.,0.,1.));
#5962=DIRECTION('ref_axis',(1.,0.,0.));
#5963=DIRECTION('center_axis',(0.,0.,1.));
#5964=DIRECTION('ref_axis',(1.,0.,0.));
#5965=DIRECTION('',(0.,0.,1.));
#5966=DIRECTION('center_axis',(0.,0.,-1.));
#5967=DIRECTION('ref_axis',(1.,0.,0.));
#5968=DIRECTION('center_axis',(0.,0.,1.));
#5969=DIRECTION('ref_axis',(1.,0.,0.));
#5970=DIRECTION('center_axis',(0.,0.,1.));
#5971=DIRECTION('ref_axis',(1.,0.,0.));
#5972=DIRECTION('',(0.,0.,1.));
#5973=DIRECTION('center_axis',(0.,0.,-1.));
#5974=DIRECTION('ref_axis',(1.,0.,0.));
#5975=DIRECTION('center_axis',(0.,0.,1.));
#5976=DIRECTION('ref_axis',(1.,0.,0.));
#5977=DIRECTION('center_axis',(0.,0.,1.));
#5978=DIRECTION('ref_axis',(1.,0.,0.));
#5979=DIRECTION('',(0.,0.,1.));
#5980=DIRECTION('center_axis',(0.,0.,-1.));
#5981=DIRECTION('ref_axis',(1.,0.,0.));
#5982=DIRECTION('center_axis',(0.,1.,0.));
#5983=DIRECTION('ref_axis',(-1.,0.,0.));
#5984=DIRECTION('',(-1.,0.,0.));
#5985=DIRECTION('',(0.,0.,1.));
#5986=DIRECTION('',(-1.,0.,0.));
#5987=DIRECTION('',(0.,0.,1.));
#5988=DIRECTION('center_axis',(1.,0.,0.));
#5989=DIRECTION('ref_axis',(0.,1.,0.));
#5990=DIRECTION('',(0.,1.,0.));
#5991=DIRECTION('',(0.,1.,0.));
#5992=DIRECTION('',(0.,0.,1.));
#5993=DIRECTION('center_axis',(0.,-1.,0.));
#5994=DIRECTION('ref_axis',(1.,0.,0.));
#5995=DIRECTION('',(1.,0.,0.));
#5996=DIRECTION('',(1.,0.,0.));
#5997=DIRECTION('',(0.,0.,1.));
#5998=DIRECTION('center_axis',(-1.,0.,0.));
#5999=DIRECTION('ref_axis',(0.,-1.,0.));
#6000=DIRECTION('',(0.,-1.,0.));
#6001=DIRECTION('',(0.,-1.,0.));
#6002=DIRECTION('center_axis',(0.,0.,1.));
#6003=DIRECTION('ref_axis',(1.,0.,0.));
#6004=DIRECTION('center_axis',(0.,0.,1.));
#6005=DIRECTION('ref_axis',(1.,0.,0.));
#7408=CARTESIAN_POINT('',(0.,0.,0.));
#7409=CARTESIAN_POINT('Origin',(11.7,-1.6,-0.1));
#7410=CARTESIAN_POINT('',(11.49,-1.6,0.));
#7411=CARTESIAN_POINT('Origin',(11.7,-1.6,0.));
#7412=CARTESIAN_POINT('',(11.49,-1.6,1.));
#7413=CARTESIAN_POINT('',(11.49,-1.6,-0.1));
#7414=CARTESIAN_POINT('Origin',(11.7,-1.6,1.));
#7415=CARTESIAN_POINT('Origin',(9.5,1.6,-0.1));
#7416=CARTESIAN_POINT('',(9.29,1.6,0.));
#7417=CARTESIAN_POINT('Origin',(9.5,1.6,0.));
#7418=CARTESIAN_POINT('',(9.29,1.6,1.));
#7419=CARTESIAN_POINT('',(9.29,1.6,-0.1));
#7420=CARTESIAN_POINT('Origin',(9.5,1.6,1.));
#7421=CARTESIAN_POINT('Origin',(9.5,-1.6,-0.1));
#7422=CARTESIAN_POINT('',(9.29,-1.6,0.));
#7423=CARTESIAN_POINT('Origin',(9.5,-1.6,0.));
#7424=CARTESIAN_POINT('',(9.29,-1.6,1.));
#7425=CARTESIAN_POINT('',(9.29,-1.6,-0.1));
#7426=CARTESIAN_POINT('Origin',(9.5,-1.6,1.));
#7427=CARTESIAN_POINT('Origin',(11.7,1.6,-0.1));
#7428=CARTESIAN_POINT('',(11.49,1.6,0.));
#7429=CARTESIAN_POINT('Origin',(11.7,1.6,0.));
#7430=CARTESIAN_POINT('',(11.49,1.6,1.));
#7431=CARTESIAN_POINT('',(11.49,1.6,-0.1));
#7432=CARTESIAN_POINT('Origin',(11.7,1.6,1.));
#7433=CARTESIAN_POINT('Origin',(26.5,-5.5,-0.1));
#7434=CARTESIAN_POINT('',(26.29,-5.5,0.));
#7435=CARTESIAN_POINT('Origin',(26.5,-5.5,0.));
#7436=CARTESIAN_POINT('',(26.29,-5.5,1.));
#7437=CARTESIAN_POINT('',(26.29,-5.5,-0.1));
#7438=CARTESIAN_POINT('Origin',(26.5,-5.5,1.));
#7439=CARTESIAN_POINT('Origin',(3.5,5.5,-0.1));
#7440=CARTESIAN_POINT('',(3.29,5.5,0.));
#7441=CARTESIAN_POINT('Origin',(3.5,5.5,0.));
#7442=CARTESIAN_POINT('',(3.29,5.5,1.));
#7443=CARTESIAN_POINT('',(3.29,5.5,-0.1));
#7444=CARTESIAN_POINT('Origin',(3.5,5.5,1.));
#7445=CARTESIAN_POINT('Origin',(3.5,-5.5,-0.1));
#7446=CARTESIAN_POINT('',(3.29,-5.5,0.));
#7447=CARTESIAN_POINT('Origin',(3.5,-5.5,0.));
#7448=CARTESIAN_POINT('',(3.29,-5.5,1.));
#7449=CARTESIAN_POINT('',(3.29,-5.5,-0.1));
#7450=CARTESIAN_POINT('Origin',(3.5,-5.5,1.));
#7451=CARTESIAN_POINT('Origin',(26.5,5.5,-0.1));
#7452=CARTESIAN_POINT('',(26.29,5.5,0.));
#7453=CARTESIAN_POINT('Origin',(26.5,5.5,0.));
#7454=CARTESIAN_POINT('',(26.29,5.5,1.));
#7455=CARTESIAN_POINT('',(26.29,5.5,-0.1));
#7456=CARTESIAN_POINT('Origin',(26.5,5.5,1.));
#7457=CARTESIAN_POINT('Origin',(29.,2.4,-0.1));
#7458=CARTESIAN_POINT('',(28.79,2.4,0.));
#7459=CARTESIAN_POINT('Origin',(29.,2.4,0.));
#7460=CARTESIAN_POINT('',(28.79,2.4,1.));
#7461=CARTESIAN_POINT('',(28.79,2.4,-0.1));
#7462=CARTESIAN_POINT('Origin',(29.,2.4,1.));
#7463=CARTESIAN_POINT('Origin',(29.,-5.6,-0.1));
#7464=CARTESIAN_POINT('',(28.79,-5.6,0.));
#7465=CARTESIAN_POINT('Origin',(29.,-5.6,0.));
#7466=CARTESIAN_POINT('',(28.79,-5.6,1.));
#7467=CARTESIAN_POINT('',(28.79,-5.6,-0.1));
#7468=CARTESIAN_POINT('Origin',(29.,-5.6,1.));
#7469=CARTESIAN_POINT('Origin',(1.,5.6,-0.1));
#7470=CARTESIAN_POINT('',(0.79,5.6,0.));
#7471=CARTESIAN_POINT('Origin',(1.,5.6,0.));
#7472=CARTESIAN_POINT('',(0.79,5.6,1.));
#7473=CARTESIAN_POINT('',(0.79,5.6,-0.1));
#7474=CARTESIAN_POINT('Origin',(1.,5.6,1.));
#7475=CARTESIAN_POINT('Origin',(1.,-2.4,-0.1));
#7476=CARTESIAN_POINT('',(0.79,-2.4,0.));
#7477=CARTESIAN_POINT('Origin',(1.,-2.4,0.));
#7478=CARTESIAN_POINT('',(0.79,-2.4,1.));
#7479=CARTESIAN_POINT('',(0.79,-2.4,-0.1));
#7480=CARTESIAN_POINT('Origin',(1.,-2.4,1.));
#7481=CARTESIAN_POINT('Origin',(1.,2.4,-0.1));
#7482=CARTESIAN_POINT('',(0.79,2.4,0.));
#7483=CARTESIAN_POINT('Origin',(1.,2.4,0.));
#7484=CARTESIAN_POINT('',(0.79,2.4,1.));
#7485=CARTESIAN_POINT('',(0.79,2.4,-0.1));
#7486=CARTESIAN_POINT('Origin',(1.,2.4,1.));
#7487=CARTESIAN_POINT('Origin',(1.,-5.6,-0.1));
#7488=CARTESIAN_POINT('',(0.79,-5.6,0.));
#7489=CARTESIAN_POINT('Origin',(1.,-5.6,0.));
#7490=CARTESIAN_POINT('',(0.79,-5.6,1.));
#7491=CARTESIAN_POINT('',(0.79,-5.6,-0.1));
#7492=CARTESIAN_POINT('Origin',(1.,-5.6,1.));
#7493=CARTESIAN_POINT('Origin',(29.,-2.4,-0.1));
#7494=CARTESIAN_POINT('',(28.79,-2.4,0.));
#7495=CARTESIAN_POINT('Origin',(29.,-2.4,0.));
#7496=CARTESIAN_POINT('',(28.79,-2.4,1.));
#7497=CARTESIAN_POINT('',(28.79,-2.4,-0.1));
#7498=CARTESIAN_POINT('Origin',(29.,-2.4,1.));
#7499=CARTESIAN_POINT('Origin',(29.,5.6,-0.1));
#7500=CARTESIAN_POINT('',(28.79,5.6,0.));
#7501=CARTESIAN_POINT('Origin',(29.,5.6,0.));
#7502=CARTESIAN_POINT('',(28.79,5.6,1.));
#7503=CARTESIAN_POINT('',(28.79,5.6,-0.1));
#7504=CARTESIAN_POINT('Origin',(29.,5.6,1.));
#7505=CARTESIAN_POINT('Origin',(31.,7.5,0.));
#7506=CARTESIAN_POINT('',(31.,7.5,0.));
#7507=CARTESIAN_POINT('',(-1.,7.5,0.));
#7508=CARTESIAN_POINT('',(31.,7.5,0.));
#7509=CARTESIAN_POINT('',(-1.,7.5,1.));
#7510=CARTESIAN_POINT('',(-1.,7.5,0.));
#7511=CARTESIAN_POINT('',(31.,7.5,1.));
#7512=CARTESIAN_POINT('',(31.,7.5,1.));
#7513=CARTESIAN_POINT('',(31.,7.5,0.));
#7514=CARTESIAN_POINT('Origin',(31.,-7.5,0.));
#7515=CARTESIAN_POINT('',(31.,-7.5,0.));
#7516=CARTESIAN_POINT('',(31.,-7.5,0.));
#7517=CARTESIAN_POINT('',(31.,-7.5,1.));
#7518=CARTESIAN_POINT('',(31.,-7.5,1.));
#7519=CARTESIAN_POINT('',(31.,-7.5,0.));
#7520=CARTESIAN_POINT('Origin',(-1.,-7.5,0.));
#7521=CARTESIAN_POINT('',(-1.,-7.5,0.));
#7522=CARTESIAN_POINT('',(-1.,-7.5,0.));
#7523=CARTESIAN_POINT('',(-1.,-7.5,1.));
#7524=CARTESIAN_POINT('',(-1.,-7.5,1.));
#7525=CARTESIAN_POINT('',(-1.,-7.5,0.));
#7526=CARTESIAN_POINT('Origin',(-1.,7.5,0.));
#7527=CARTESIAN_POINT('',(-1.,7.5,0.));
#7528=CARTESIAN_POINT('',(-1.,7.5,1.));
#7529=CARTESIAN_POINT('Origin',(15.,0.,1.));
#7530=CARTESIAN_POINT('Origin',(15.,0.,0.));
#10239=UNCERTAINTY_MEASURE_WITH_UNIT(LENGTH_MEASURE(0.001),#10293,
'DISTANCE_ACCURACY_VALUE',
'Maximum model space distance between geometric entities at asserted c
onnectivities');
#10264=UNCERTAINTY_MEASURE_WITH_UNIT(LENGTH_MEASURE(0.001),#10293,
'DISTANCE_ACCURACY_VALUE',
'Maximum model space distance between geometric entities at asserted c
onnectivities');
#10267=(
GEOMETRIC_REPRESENTATION_CONTEXT(3)
GLOBAL_UNCERTAINTY_ASSIGNED_CONTEXT((#10239))
GLOBAL_UNIT_ASSIGNED_CONTEXT((#10293,#10295,#10296))
REPRESENTATION_CONTEXT('','3D')
);
#10292=(
GEOMETRIC_REPRESENTATION_CONTEXT(3)
GLOBAL_UNCERTAINTY_ASSIGNED_CONTEXT((#10264))
GLOBAL_UNIT_ASSIGNED_CONTEXT((#10293,#10295,#10296))
REPRESENTATION_CONTEXT('','3D')
);
#10293=(
LENGTH_UNIT()
NAMED_UNIT(*)
SI_UNIT(.CENTI.,.METRE.)
);
#10295=(
NAMED_UNIT(*)
PLANE_ANGLE_UNIT()
SI_UNIT($,.RADIAN.)
);
#10296=(
NAMED_UNIT(*)
SI_UNIT($,.STERADIAN.)
SOLID_ANGLE_UNIT()
);
#10299=SHAPE_DEFINITION_REPRESENTATION(#10326,#10415);
#10326=PRODUCT_DEFINITION_SHAPE('',$,#10443);
#10415=SHAPE_REPRESENTATION('',(#5291),#10267);
#10440=PRODUCT_DEFINITION_CONTEXT('part definition',#10523,'design');
#10443=PRODUCT_DEFINITION('Stop-mounted base plate',
'Stop-mounted base plate',#10470,#10440);
#10470=PRODUCT_DEFINITION_FORMATION('',$,#10527);
#10523=APPLICATION_CONTEXT(
'Core Data for Automotive Mechanical Design Process');
#10524=PRODUCT_CONTEXT('part definition',#10523,'mechanical');
#10527=PRODUCT('Stop-mounted base plate','Stop-mounted base plate','Stop-mounted base plate',(#10524));
#10601=COLOUR_RGB('Dark Blue',0.08,0.2,0.34);
#10602=FILL_AREA_STYLE_COLOUR('',#10601);
#10603=FILL_AREA_STYLE('',(#10602));
#10604=SURFACE_STYLE_FILL_AREA(#10603);
#10605=SURFACE_SIDE_STYLE('',(#10604));
#10606=SURFACE_STYLE_USAGE(.BOTH.,#10605);
#10607=PRESENTATION_STYLE_ASSIGNMENT((#10606));
ENDSEC;
END-ISO-10303-21;
